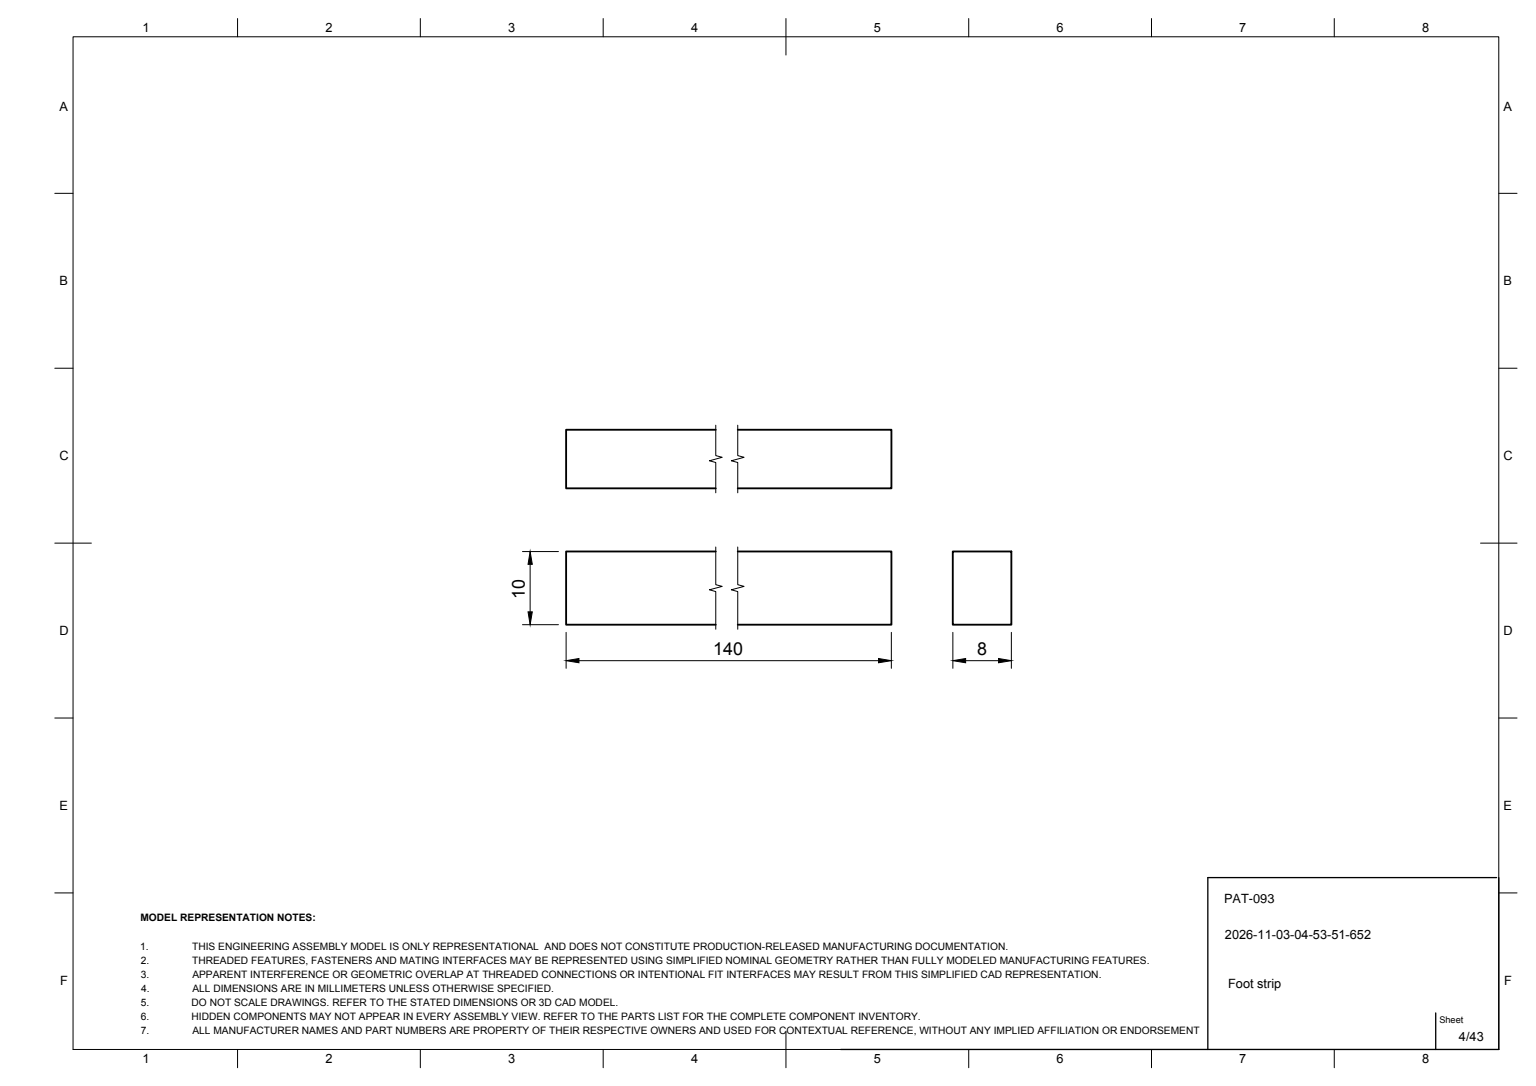
ISO-10303-21;
HEADER;
/* Generated by software containing ST-Developer
 * from STEP Tools, Inc. (www.steptools.com) 
 */

FILE_DESCRIPTION(
/* description */ ('Self-centering screw clamp'),
/* implementation_level */ '2;1');

FILE_NAME(
/* name */ 'Foot strip.step',
/* time_stamp */ '2026-10-28T03:25:31-07:00',
/* author */ (''),
/* organization */ (''),
/* preprocessor_version */ 'ST-DEVELOPER v20.2',
/* originating_system */ 'Autodesk Translation Framework v15.17.0.0',
/* authorisation */ '');

FILE_SCHEMA (('AUTOMOTIVE_DESIGN { 1 0 10303 214 3 1 1 }'));
ENDSEC;

DATA;
#10=MECHANICAL_DESIGN_GEOMETRIC_PRESENTATION_REPRESENTATION('',(#625),#16799);
#543=SHAPE_REPRESENTATION_RELATIONSHIP('SRR','None',#17016,#584);
#584=ADVANCED_BREP_SHAPE_REPRESENTATION('',(#673),#16754);
#625=STYLED_ITEM('',(#17312),#673);
#673=MANIFOLD_SOLID_BREP('Body1',#9076);
#1020=PLANE('',#9623);
#1021=PLANE('',#9624);
#1022=PLANE('',#9625);
#1023=PLANE('',#9626);
#1024=PLANE('',#9627);
#1025=PLANE('',#9628);
#1291=FACE_OUTER_BOUND('',#1819,.T.);
#1292=FACE_OUTER_BOUND('',#1820,.T.);
#1293=FACE_OUTER_BOUND('',#1821,.T.);
#1294=FACE_OUTER_BOUND('',#1822,.T.);
#1295=FACE_OUTER_BOUND('',#1823,.T.);
#1296=FACE_OUTER_BOUND('',#1824,.T.);
#1819=EDGE_LOOP('',(#6199,#6200,#6201,#6202));
#1820=EDGE_LOOP('',(#6203,#6204,#6205,#6206));
#1821=EDGE_LOOP('',(#6207,#6208,#6209,#6210));
#1822=EDGE_LOOP('',(#6211,#6212,#6213,#6214));
#1823=EDGE_LOOP('',(#6215,#6216,#6217,#6218));
#1824=EDGE_LOOP('',(#6219,#6220,#6221,#6222));
#2601=LINE('',#13780,#3174);
#2602=LINE('',#13782,#3175);
#2603=LINE('',#13784,#3176);
#2604=LINE('',#13785,#3177);
#2605=LINE('',#13788,#3178);
#2606=LINE('',#13790,#3179);
#2607=LINE('',#13791,#3180);
#2608=LINE('',#13794,#3181);
#2609=LINE('',#13796,#3182);
#2610=LINE('',#13797,#3183);
#2611=LINE('',#13799,#3184);
#2612=LINE('',#13800,#3185);
#3174=VECTOR('',#10870,1.);
#3175=VECTOR('',#10871,1.);
#3176=VECTOR('',#10872,1.);
#3177=VECTOR('',#10873,1.);
#3178=VECTOR('',#10876,1.);
#3179=VECTOR('',#10877,1.);
#3180=VECTOR('',#10878,1.);
#3181=VECTOR('',#10881,1.);
#3182=VECTOR('',#10882,1.);
#3183=VECTOR('',#10883,1.);
#3184=VECTOR('',#10886,1.);
#3185=VECTOR('',#10887,1.);
#4265=VERTEX_POINT('',#13778);
#4266=VERTEX_POINT('',#13779);
#4267=VERTEX_POINT('',#13781);
#4268=VERTEX_POINT('',#13783);
#4269=VERTEX_POINT('',#13787);
#4270=VERTEX_POINT('',#13789);
#4271=VERTEX_POINT('',#13793);
#4272=VERTEX_POINT('',#13795);
#5024=EDGE_CURVE('',#4265,#4266,#2601,.T.);
#5025=EDGE_CURVE('',#4266,#4267,#2602,.T.);
#5026=EDGE_CURVE('',#4268,#4267,#2603,.T.);
#5027=EDGE_CURVE('',#4265,#4268,#2604,.T.);
#5028=EDGE_CURVE('',#4269,#4265,#2605,.T.);
#5029=EDGE_CURVE('',#4270,#4268,#2606,.T.);
#5030=EDGE_CURVE('',#4269,#4270,#2607,.T.);
#5031=EDGE_CURVE('',#4271,#4269,#2608,.T.);
#5032=EDGE_CURVE('',#4272,#4270,#2609,.T.);
#5033=EDGE_CURVE('',#4271,#4272,#2610,.T.);
#5034=EDGE_CURVE('',#4266,#4271,#2611,.T.);
#5035=EDGE_CURVE('',#4267,#4272,#2612,.T.);
#6199=ORIENTED_EDGE('',*,*,#5024,.T.);
#6200=ORIENTED_EDGE('',*,*,#5025,.T.);
#6201=ORIENTED_EDGE('',*,*,#5026,.F.);
#6202=ORIENTED_EDGE('',*,*,#5027,.F.);
#6203=ORIENTED_EDGE('',*,*,#5028,.T.);
#6204=ORIENTED_EDGE('',*,*,#5027,.T.);
#6205=ORIENTED_EDGE('',*,*,#5029,.F.);
#6206=ORIENTED_EDGE('',*,*,#5030,.F.);
#6207=ORIENTED_EDGE('',*,*,#5031,.T.);
#6208=ORIENTED_EDGE('',*,*,#5030,.T.);
#6209=ORIENTED_EDGE('',*,*,#5032,.F.);
#6210=ORIENTED_EDGE('',*,*,#5033,.F.);
#6211=ORIENTED_EDGE('',*,*,#5034,.T.);
#6212=ORIENTED_EDGE('',*,*,#5033,.T.);
#6213=ORIENTED_EDGE('',*,*,#5035,.F.);
#6214=ORIENTED_EDGE('',*,*,#5025,.F.);
#6215=ORIENTED_EDGE('',*,*,#5035,.T.);
#6216=ORIENTED_EDGE('',*,*,#5032,.T.);
#6217=ORIENTED_EDGE('',*,*,#5029,.T.);
#6218=ORIENTED_EDGE('',*,*,#5026,.T.);
#6219=ORIENTED_EDGE('',*,*,#5034,.F.);
#6220=ORIENTED_EDGE('',*,*,#5024,.F.);
#6221=ORIENTED_EDGE('',*,*,#5028,.F.);
#6222=ORIENTED_EDGE('',*,*,#5031,.F.);
#8589=ADVANCED_FACE('',(#1291),#1020,.T.);
#8590=ADVANCED_FACE('',(#1292),#1021,.T.);
#8591=ADVANCED_FACE('',(#1293),#1022,.T.);
#8592=ADVANCED_FACE('',(#1294),#1023,.T.);
#8593=ADVANCED_FACE('',(#1295),#1024,.T.);
#8594=ADVANCED_FACE('',(#1296),#1025,.F.);
#9076=CLOSED_SHELL('',(#8589,#8590,#8591,#8592,#8593,#8594));
#9622=AXIS2_PLACEMENT_3D('',#13776,#10866,#10867);
#9623=AXIS2_PLACEMENT_3D('',#13777,#10868,#10869);
#9624=AXIS2_PLACEMENT_3D('',#13786,#10874,#10875);
#9625=AXIS2_PLACEMENT_3D('',#13792,#10879,#10880);
#9626=AXIS2_PLACEMENT_3D('',#13798,#10884,#10885);
#9627=AXIS2_PLACEMENT_3D('',#13801,#10888,#10889);
#9628=AXIS2_PLACEMENT_3D('',#13802,#10890,#10891);
#10866=DIRECTION('axis',(0.,0.,1.));
#10867=DIRECTION('refdir',(1.,0.,0.));
#10868=DIRECTION('center_axis',(0.,1.,0.));
#10869=DIRECTION('ref_axis',(-1.,0.,0.));
#10870=DIRECTION('',(-1.,0.,0.));
#10871=DIRECTION('',(0.,0.,1.));
#10872=DIRECTION('',(-1.,0.,0.));
#10873=DIRECTION('',(0.,0.,1.));
#10874=DIRECTION('center_axis',(1.,0.,0.));
#10875=DIRECTION('ref_axis',(0.,1.,0.));
#10876=DIRECTION('',(0.,1.,0.));
#10877=DIRECTION('',(0.,1.,0.));
#10878=DIRECTION('',(0.,0.,1.));
#10879=DIRECTION('center_axis',(0.,-1.,0.));
#10880=DIRECTION('ref_axis',(1.,0.,0.));
#10881=DIRECTION('',(1.,0.,0.));
#10882=DIRECTION('',(1.,0.,0.));
#10883=DIRECTION('',(0.,0.,1.));
#10884=DIRECTION('center_axis',(-1.,0.,0.));
#10885=DIRECTION('ref_axis',(0.,-1.,0.));
#10886=DIRECTION('',(0.,-1.,0.));
#10887=DIRECTION('',(0.,-1.,0.));
#10888=DIRECTION('center_axis',(0.,0.,1.));
#10889=DIRECTION('ref_axis',(1.,0.,0.));
#10890=DIRECTION('center_axis',(0.,0.,1.));
#10891=DIRECTION('ref_axis',(1.,0.,0.));
#13776=CARTESIAN_POINT('',(0.,0.,0.));
#13777=CARTESIAN_POINT('Origin',(-15.,7.,-0.8));
#13778=CARTESIAN_POINT('',(-15.,7.,-0.8));
#13779=CARTESIAN_POINT('',(-16.,7.,-0.8));
#13780=CARTESIAN_POINT('',(-15.,7.,-0.8));
#13781=CARTESIAN_POINT('',(-16.,7.,0.));
#13782=CARTESIAN_POINT('',(-16.,7.,-0.8));
#13783=CARTESIAN_POINT('',(-15.,7.,0.));
#13784=CARTESIAN_POINT('',(-15.,7.,0.));
#13785=CARTESIAN_POINT('',(-15.,7.,-0.8));
#13786=CARTESIAN_POINT('Origin',(-15.,-7.,-0.8));
#13787=CARTESIAN_POINT('',(-15.,-7.,-0.8));
#13788=CARTESIAN_POINT('',(-15.,-7.,-0.8));
#13789=CARTESIAN_POINT('',(-15.,-7.,0.));
#13790=CARTESIAN_POINT('',(-15.,-7.,0.));
#13791=CARTESIAN_POINT('',(-15.,-7.,-0.8));
#13792=CARTESIAN_POINT('Origin',(-16.,-7.,-0.8));
#13793=CARTESIAN_POINT('',(-16.,-7.,-0.8));
#13794=CARTESIAN_POINT('',(-16.,-7.,-0.8));
#13795=CARTESIAN_POINT('',(-16.,-7.,0.));
#13796=CARTESIAN_POINT('',(-16.,-7.,0.));
#13797=CARTESIAN_POINT('',(-16.,-7.,-0.8));
#13798=CARTESIAN_POINT('Origin',(-16.,7.,-0.8));
#13799=CARTESIAN_POINT('',(-16.,7.,-0.8));
#13800=CARTESIAN_POINT('',(-16.,7.,0.));
#13801=CARTESIAN_POINT('Origin',(-15.5,0.,0.));
#13802=CARTESIAN_POINT('Origin',(-15.5,0.,-0.8));
#16705=UNCERTAINTY_MEASURE_WITH_UNIT(LENGTH_MEASURE(0.001),#16800,
'DISTANCE_ACCURACY_VALUE',
'Maximum model space distance between geometric entities at asserted c
onnectivities');
#16750=UNCERTAINTY_MEASURE_WITH_UNIT(LENGTH_MEASURE(0.001),#16800,
'DISTANCE_ACCURACY_VALUE',
'Maximum model space distance between geometric entities at asserted c
onnectivities');
#16754=(
GEOMETRIC_REPRESENTATION_CONTEXT(3)
GLOBAL_UNCERTAINTY_ASSIGNED_CONTEXT((#16705))
GLOBAL_UNIT_ASSIGNED_CONTEXT((#16800,#16802,#16803))
REPRESENTATION_CONTEXT('','3D')
);
#16799=(
GEOMETRIC_REPRESENTATION_CONTEXT(3)
GLOBAL_UNCERTAINTY_ASSIGNED_CONTEXT((#16750))
GLOBAL_UNIT_ASSIGNED_CONTEXT((#16800,#16802,#16803))
REPRESENTATION_CONTEXT('','3D')
);
#16800=(
LENGTH_UNIT()
NAMED_UNIT(*)
SI_UNIT(.CENTI.,.METRE.)
);
#16802=(
NAMED_UNIT(*)
PLANE_ANGLE_UNIT()
SI_UNIT($,.RADIAN.)
);
#16803=(
NAMED_UNIT(*)
SI_UNIT($,.STERADIAN.)
SOLID_ANGLE_UNIT()
);
#16807=SHAPE_DEFINITION_REPRESENTATION(#16855,#17016);
#16855=PRODUCT_DEFINITION_SHAPE('',$,#17065);
#17016=SHAPE_REPRESENTATION('',(#9622),#16754);
#17061=PRODUCT_DEFINITION_CONTEXT('part definition',#17207,'design');
#17065=PRODUCT_DEFINITION('Foot strip','Foot strip',#17113,#17061);
#17113=PRODUCT_DEFINITION_FORMATION('',$,#17212);
#17207=APPLICATION_CONTEXT(
'Core Data for Automotive Mechanical Design Process');
#17208=PRODUCT_CONTEXT('part definition',#17207,'mechanical');
#17212=PRODUCT('Foot strip','Foot strip','Foot strip',(#17208));
#17306=COLOUR_RGB('Light Blue',0.38,0.62,0.78);
#17307=FILL_AREA_STYLE_COLOUR('',#17306);
#17308=FILL_AREA_STYLE('',(#17307));
#17309=SURFACE_STYLE_FILL_AREA(#17308);
#17310=SURFACE_SIDE_STYLE('',(#17309));
#17311=SURFACE_STYLE_USAGE(.BOTH.,#17310);
#17312=PRESENTATION_STYLE_ASSIGNMENT((#17311));
ENDSEC;
END-ISO-10303-21;
